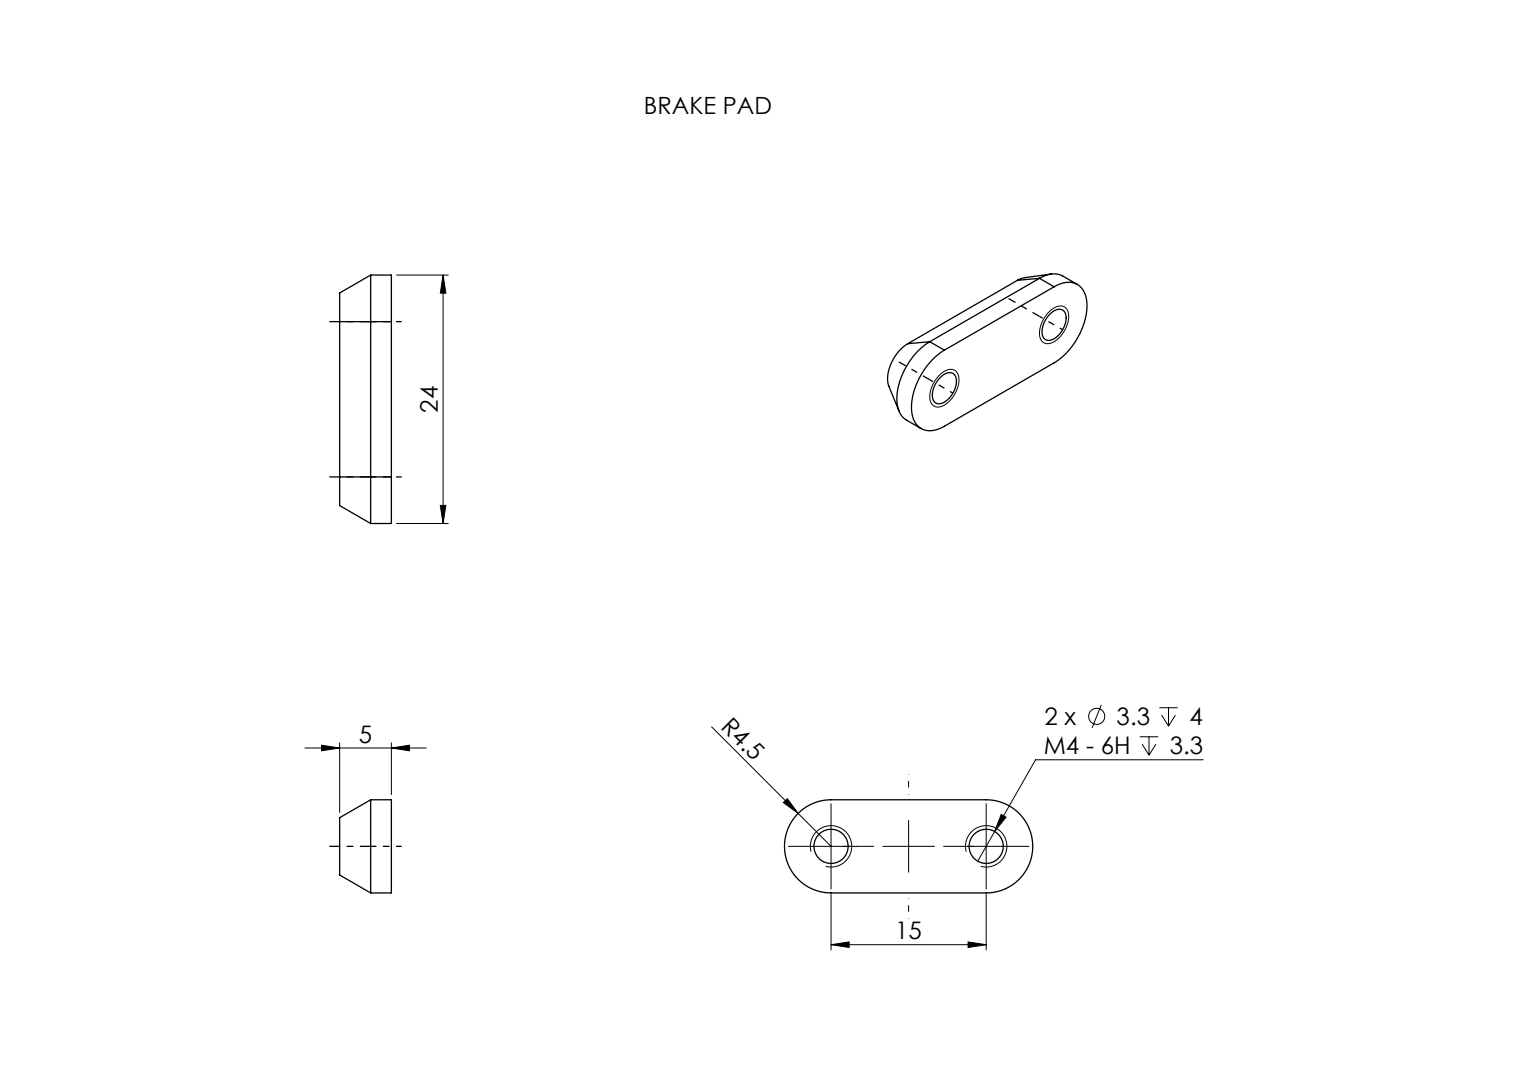
ISO-10303-21;
HEADER;
FILE_DESCRIPTION (('STEP AP214'),
    '1' );
FILE_NAME ('brake pad.step',
    '2026-10-08T05:45:04',
    ( '' ),
    ( '' ),
    'SwSTEP 2.0',
    'SolidWorks 2026',
    '' );
FILE_SCHEMA (( 'AUTOMOTIVE_DESIGN' ));
ENDSEC;

DATA;
#2=( LENGTH_UNIT ( ) NAMED_UNIT ( * ) SI_UNIT ( .MILLI., .METRE. ) );
#24=LINE ( 'NONE', #3426, #7602 ) ;
#25=FACE_OUTER_BOUND ( 'NONE', #10724, .T. ) ;
#72=( GEOMETRIC_REPRESENTATION_CONTEXT ( 3 ) GLOBAL_UNCERTAINTY_ASSIGNED_CONTEXT ( ( #3080 ) ) GLOBAL_UNIT_ASSIGNED_CONTEXT ( ( #8638, #7131, #1020 ) ) REPRESENTATION_CONTEXT ( 'NONE', 'WORKASPACE' ) );
#75=SHAPE_REPRESENTATION ( 'brake pad', ( #308 ), #6353 ) ;
#80=CARTESIAN_POINT ( 'NONE',  ( 24.49999999999999289, -3.999999999999986233, -4.999999999999992006 ) ) ;
#87=ADVANCED_FACE ( 'NONE', ( #5248 ), #2694, .F. ) ;
#161=ORIENTED_EDGE ( 'NONE', *, *, #5009, .F. ) ;
#193=ORIENTED_EDGE ( 'NONE', *, *, #720, .T. ) ;
#218=PRODUCT ( 'brake pad', 'brake pad', '', ( #1890 ) ) ;
#221=CIRCLE ( 'NONE', #5903, 1.649999999999998579 ) ;
#252=CONICAL_SURFACE ( 'NONE', #4877, 2.767949192431121919, 0.5235987755982963732 ) ;
#259=AXIS2_PLACEMENT_3D ( 'NONE', #6737, #6069, #4302 ) ;
#274=VECTOR ( 'NONE', #6744, 1000.000000000000000 ) ;
#281=VERTEX_POINT ( 'NONE', #1064 ) ;
#301=CARTESIAN_POINT ( 'NONE',  ( 24.49999999999999289, -3.999999999999986233, -9.499999999999991118 ) ) ;
#303=ORIENTED_EDGE ( 'NONE', *, *, #5009, .T. ) ;
#308=AXIS2_PLACEMENT_3D ( 'NONE', #6956, #4296, #9565 ) ;
#314=CARTESIAN_POINT ( 'NONE',  ( 27.50000000000001066, 0.5000000000000162093, 10.00000000000000888 ) ) ;
#336=FILL_AREA_STYLE ('',( #9671 ) ) ;
#356=FACE_OUTER_BOUND ( 'NONE', #2898, .T. ) ;
#358=EDGE_CURVE ( 'NONE', #6966, #10495, #2017, .T. ) ;
#363=DIRECTION ( 'NONE',  ( 0.000000000000000000, 0.000000000000000000, -1.000000000000000000 ) ) ;
#366=ORIENTED_EDGE ( 'NONE', *, *, #5633, .F. ) ;
#372=EDGE_CURVE ( 'NONE', #1417, #4847, #7538, .T. ) ;
#414=FACE_OUTER_BOUND ( 'NONE', #5327, .T. ) ;
#418=EDGE_CURVE ( 'NONE', #6185, #829, #4717, .T. ) ;
#431=ORIENTED_EDGE ( 'NONE', *, *, #9265, .T. ) ;
#465=CARTESIAN_POINT ( 'NONE',  ( 27.50000000000001066, -8.499999999999985789, -4.999999999999992006 ) ) ;
#486=EDGE_LOOP ( 'NONE', ( #10969, #5668, #5395 ) ) ;
#531=EDGE_LOOP ( 'NONE', ( #5767, #5211, #193 ) ) ;
#594=EDGE_LOOP ( 'NONE', ( #6389, #7026, #1992, #1296 ) ) ;
#605=CIRCLE ( 'NONE', #5598, 4.499999999999999112 ) ;
#653=DIRECTION ( 'NONE',  ( 1.000000000000000000, -0.000000000000000000, 1.156482317317871478E-16 ) ) ;
#675=CARTESIAN_POINT ( 'NONE',  ( 25.49999999999999645, -3.999999999999986233, -6.649999999999990585 ) ) ;
#686=LINE ( 'NONE', #7469, #1983 ) ;
#707=CARTESIAN_POINT ( 'NONE',  ( 27.50000000000001066, -3.999999999999986233, -4.999999999999992006 ) ) ;
#720=EDGE_CURVE ( 'NONE', #2294, #2160, #221, .T. ) ;
#723=DIRECTION ( 'NONE',  ( 1.000000000000000000, 0.000000000000000000, 0.000000000000000000 ) ) ;
#740=EDGE_CURVE ( 'NONE', #7218, #1417, #8677, .T. ) ;
#774=CIRCLE ( 'NONE', #5758, 4.499999999999999112 ) ;
#829=VERTEX_POINT ( 'NONE', #10864 ) ;
#848=CARTESIAN_POINT ( 'NONE',  ( 25.49999999999999645, -3.999999999999986233, -3.349999999999993427 ) ) ;
#860=DIRECTION ( 'NONE',  ( -1.156482317317871478E-16, 1.807003620809174139E-16, 1.000000000000000000 ) ) ;
#884=CARTESIAN_POINT ( 'NONE',  ( 25.49999999999999645, -3.999999999999983569, 10.00000000000000888 ) ) ;
#931=SHAPE_DEFINITION_REPRESENTATION ( #7149, #75 ) ;
#938=ADVANCED_FACE ( 'NONE', ( #10453 ), #10282, .T. ) ;
#967=AXIS2_PLACEMENT_3D ( 'NONE', #10328, #5168, #10996 ) ;
#969=DIRECTION ( 'NONE',  ( -1.156482317317871478E-16, 0.000000000000000000, 1.000000000000000000 ) ) ;
#993=CARTESIAN_POINT ( 'NONE',  ( 24.49999999999999289, -3.999999999999986233, -7.767949192431114369 ) ) ;
#997=DIRECTION ( 'NONE',  ( 0.000000000000000000, 0.000000000000000000, -1.000000000000000000 ) ) ;
#1020=( NAMED_UNIT ( * ) SI_UNIT ( $, .STERADIAN. ) SOLID_ANGLE_UNIT ( ) );
#1029=COLOUR_RGB ( '', 0.66274510, 0.83137255, 0.94901961) ;
#1036=AXIS2_PLACEMENT_3D ( 'NONE', #884, #10173, #2562 ) ;
#1038=DIRECTION ( 'NONE',  ( 0.5150380749100551547, 0.000000000000000000, -0.8571673007021116675 ) ) ;
#1064=CARTESIAN_POINT ( 'NONE',  ( 29.49999999999999645, -3.999999999999986233, -6.649999999999981704 ) ) ;
#1081=CIRCLE ( 'NONE', #4649, 2.767949192431121919 ) ;
#1153=ORIENTED_EDGE ( 'NONE', *, *, #10578, .F. ) ;
#1196=VECTOR ( 'NONE', #9291, 1000.000000000000000 ) ;
#1217=VECTOR ( 'NONE', #7964, 1000.000000000000114 ) ;
#1232=ADVANCED_BREP_SHAPE_REPRESENTATION ( '', ( #8973, #308 ), #6353 ) ;
#1245=DIRECTION ( 'NONE',  ( 0.000000000000000000, 0.000000000000000000, -1.000000000000000000 ) ) ;
#1275=DIRECTION ( 'NONE',  ( 1.000000000000000000, 6.098637220230963674E-17, 1.156482317317871478E-16 ) ) ;
#1288=VECTOR ( 'NONE', #2104, 1000.000000000000000 ) ;
#1289=EDGE_CURVE ( 'NONE', #829, #1417, #3766, .T. ) ;
#1296=ORIENTED_EDGE ( 'NONE', *, *, #9131, .F. ) ;
#1301=CARTESIAN_POINT ( 'NONE',  ( 29.49999999999999645, 0.5000000000000135447, -4.999999999999991118 ) ) ;
#1321=ADVANCED_FACE ( 'NONE', ( #414 ), #7150, .F. ) ;
#1334=VERTEX_POINT ( 'NONE', #314 ) ;
#1395=DIRECTION ( 'NONE',  ( 0.000000000000000000, 0.000000000000000000, 1.000000000000000000 ) ) ;
#1417=VERTEX_POINT ( 'NONE', #5545 ) ;
#1485=ORIENTED_EDGE ( 'NONE', *, *, #1289, .F. ) ;
#1496=VECTOR ( 'NONE', #2306, 1000.000000000000000 ) ;
#1541=VECTOR ( 'NONE', #2747, 1000.000000000000000 ) ;
#1555=CARTESIAN_POINT ( 'NONE',  ( 29.49999999999999645, -3.999999999999986233, -3.350000000000001421 ) ) ;
#1655=ORIENTED_EDGE ( 'NONE', *, *, #4757, .T. ) ;
#1686=CARTESIAN_POINT ( 'NONE',  ( 29.49999999999999645, -3.999999999999983569, 8.350000000000013856 ) ) ;
#1692=FACE_OUTER_BOUND ( 'NONE', #531, .T. ) ;
#1695=CONICAL_SURFACE ( 'NONE', #2228, 1.649999999999998579, 1.029744258676653423 ) ;
#1708=CARTESIAN_POINT ( 'NONE',  ( 29.49999999999999645, -3.999999999999983569, 11.64999999999999858 ) ) ;
#1725=ADVANCED_FACE ( 'NONE', ( #10146 ), #1763, .T. ) ;
#1727=FACE_OUTER_BOUND ( 'NONE', #10304, .T. ) ;
#1743=( GEOMETRIC_REPRESENTATION_CONTEXT ( 3 ) GLOBAL_UNCERTAINTY_ASSIGNED_CONTEXT ( ( #9535 ) ) GLOBAL_UNIT_ASSIGNED_CONTEXT ( ( #5567, #3731, #4682 ) ) REPRESENTATION_CONTEXT ( 'NONE', 'WORKASPACE' ) );
#1745=DIRECTION ( 'NONE',  ( 0.000000000000000000, 0.000000000000000000, -1.000000000000000000 ) ) ;
#1763=PLANE ( 'NONE',  #7963 ) ;
#1764=DIRECTION ( 'NONE',  ( 0.000000000000000000, 2.312964634635742464E-16, 1.000000000000000000 ) ) ;
#1769=EDGE_CURVE ( 'NONE', #4847, #3729, #24, .T. ) ;
#1854=ORIENTED_EDGE ( 'NONE', *, *, #4757, .F. ) ;
#1890=PRODUCT_CONTEXT ( 'NONE', #3230, 'mechanical' ) ;
#1901=DIRECTION ( 'NONE',  ( -0.8660254037844401509, 0.4999999999999974465, 0.000000000000000000 ) ) ;
#1911=DIRECTION ( 'NONE',  ( 0.000000000000000000, 0.000000000000000000, -1.000000000000000000 ) ) ;
#1914=DIRECTION ( 'NONE',  ( 0.000000000000000000, 0.000000000000000000, 1.000000000000000000 ) ) ;
#1915=CARTESIAN_POINT ( 'NONE',  ( 24.49999999999999289, -8.499999999999985789, -4.999999999999992006 ) ) ;
#1929=DIRECTION ( 'NONE',  ( -1.000000000000000000, -6.098637220230963674E-17, -1.156482317317871478E-16 ) ) ;
#1972=EDGE_CURVE ( 'NONE', #2160, #2294, #6718, .T. ) ;
#1983=VECTOR ( 'NONE', #10089, 1000.000000000000000 ) ;
#1992=ORIENTED_EDGE ( 'NONE', *, *, #4028, .T. ) ;
#1994=CARTESIAN_POINT ( 'NONE',  ( 27.50000000000001066, -8.499999999999984013, 10.00000000000001243 ) ) ;
#2015=ADVANCED_FACE ( 'NONE', ( #1727 ), #3351, .F. ) ;
#2017=LINE ( 'NONE', #1915, #5074 ) ;
#2062=LINE ( 'NONE', #7164, #5810 ) ;
#2072=AXIS2_PLACEMENT_3D ( 'NONE', #9436, #3758, #4652 ) ;
#2085=LINE ( 'NONE', #1301, #5488 ) ;
#2089=EDGE_CURVE ( 'NONE', #2779, #3903, #2085, .T. ) ;
#2104=DIRECTION ( 'NONE',  ( -1.156482317317871725E-16, 2.312964634635742464E-16, 1.000000000000000000 ) ) ;
#2133=ORIENTED_EDGE ( 'NONE', *, *, #2996, .T. ) ;
#2136=CARTESIAN_POINT ( 'NONE',  ( 27.50000000000000711, 0.5000000000000162093, 10.00000000000000888 ) ) ;
#2140=DIRECTION ( 'NONE',  ( 0.000000000000000000, 0.000000000000000000, -1.000000000000000000 ) ) ;
#2141=DIRECTION ( 'NONE',  ( 1.000000000000000000, -0.000000000000000000, 1.156482317317871478E-16 ) ) ;
#2160=VERTEX_POINT ( 'NONE', #3746 ) ;
#2184=DIRECTION ( 'NONE',  ( -1.000000000000000000, -6.098637220230963674E-17, -1.156482317317871478E-16 ) ) ;
#2228=AXIS2_PLACEMENT_3D ( 'NONE', #7641, #3363, #9240 ) ;
#2231=CARTESIAN_POINT ( 'NONE',  ( 24.49999999999999289, -3.999999999999986233, -4.999999999999992006 ) ) ;
#2242=DIRECTION ( 'NONE',  ( 0.000000000000000000, 0.000000000000000000, 1.000000000000000000 ) ) ;
#2251=AXIS2_PLACEMENT_3D ( 'NONE', #10250, #4308, #6026 ) ;
#2268=EDGE_CURVE ( 'NONE', #3729, #6185, #1081, .T. ) ;
#2294=VERTEX_POINT ( 'NONE', #675 ) ;
#2297=CARTESIAN_POINT ( 'NONE',  ( 24.49999999999999289, -8.499999999999985789, -4.999999999999992006 ) ) ;
#2306=DIRECTION ( 'NONE',  ( 1.000000000000000000, 6.098637220230963674E-17, 1.156482317317871478E-16 ) ) ;
#2331=ADVANCED_FACE ( 'NONE', ( #10074 ), #6055, .T. ) ;
#2360=ADVANCED_FACE ( 'NONE', ( #4245 ), #3127, .F. ) ;
#2376=ORIENTED_EDGE ( 'NONE', *, *, #4928, .T. ) ;
#2377=LINE ( 'NONE', #7492, #3098 ) ;
#2403=DIRECTION ( 'NONE',  ( -1.000000000000000000, -6.098637220230963674E-17, -1.156482317317871478E-16 ) ) ;
#2414=DIRECTION ( 'NONE',  ( 1.000000000000000000, -0.000000000000000000, 1.156482317317871478E-16 ) ) ;
#2461=ORIENTED_EDGE ( 'NONE', *, *, #2089, .F. ) ;
#2526=AXIS2_PLACEMENT_3D ( 'NONE', #10493, #8926, #363 ) ;
#2532=DIRECTION ( 'NONE',  ( -0.4999999999999978906, 0.8660254037844399289, -2.143152199010143228E-16 ) ) ;
#2538=CARTESIAN_POINT ( 'NONE',  ( 29.49999999999999645, -3.999999999999986233, -9.499999999999991118 ) ) ;
#2539=EDGE_CURVE ( 'NONE', #9740, #10159, #686, .T. ) ;
#2562=DIRECTION ( 'NONE',  ( 0.000000000000000000, 0.000000000000000000, -1.000000000000000000 ) ) ;
#2565=ORIENTED_EDGE ( 'NONE', *, *, #3436, .T. ) ;
#2567=ORIENTED_EDGE ( 'NONE', *, *, #418, .T. ) ;
#2601=CARTESIAN_POINT ( 'NONE',  ( 24.50857997860451931, -3.999999999999987121, -4.999999999999992006 ) ) ;
#2623=EDGE_CURVE ( 'NONE', #9740, #5796, #6861, .T. ) ;
#2668=EDGE_LOOP ( 'NONE', ( #5565, #9709, #10121, #7284 ) ) ;
#2678=DIRECTION ( 'NONE',  ( 0.000000000000000000, 0.000000000000000000, -1.000000000000000000 ) ) ;
#2688=ADVANCED_FACE ( 'NONE', ( #9748 ), #6356, .F. ) ;
#2694=CYLINDRICAL_SURFACE ( 'NONE', #259, 1.649999999999995248 ) ;
#2706=ADVANCED_FACE ( 'NONE', ( #8866 ), #5178, .T. ) ;
#2747=DIRECTION ( 'NONE',  ( 0.5150380749100549327, 1.049727191138617956E-16, 0.8571673007021118895 ) ) ;
#2754=CARTESIAN_POINT ( 'NONE',  ( 29.49999999999999645, -3.999999999999986233, -4.999999999999991118 ) ) ;
#2779=VERTEX_POINT ( 'NONE', #3908 ) ;
#2780=ORIENTED_EDGE ( 'NONE', *, *, #8807, .T. ) ;
#2814=PRESENTATION_STYLE_ASSIGNMENT (( #4529 ) ) ;
#2816=CARTESIAN_POINT ( 'NONE',  ( 27.50000000000001066, -3.999999999999986233, -9.499999999999991118 ) ) ;
#2822=CARTESIAN_POINT ( 'NONE',  ( 29.49999999999999645, -3.999999999999983569, 10.00000000000000888 ) ) ;
#2886=ORIENTED_EDGE ( 'NONE', *, *, #10498, .T. ) ;
#2898=EDGE_LOOP ( 'NONE', ( #4680, #4279, #4909, #1485 ) ) ;
#2943=EDGE_CURVE ( 'NONE', #9728, #2779, #4480, .T. ) ;
#2986=ORIENTED_EDGE ( 'NONE', *, *, #1972, .F. ) ;
#2996=EDGE_CURVE ( 'NONE', #5796, #10159, #3585, .T. ) ;
#3080=UNCERTAINTY_MEASURE_WITH_UNIT (LENGTH_MEASURE( 1.000000000000000082E-05 ), #8638, 'distance_accuracy_value', 'NONE');
#3089=EDGE_CURVE ( 'NONE', #7474, #2294, #5274, .T. ) ;
#3098=VECTOR ( 'NONE', #653, 1000.000000000000000 ) ;
#3108=ORIENTED_EDGE ( 'NONE', *, *, #720, .F. ) ;
#3110=ORIENTED_EDGE ( 'NONE', *, *, #2623, .F. ) ;
#3127=PLANE ( 'NONE',  #8017 ) ;
#3162=CARTESIAN_POINT ( 'NONE',  ( 24.49999999999999289, -3.999999999999986233, -4.999999999999992006 ) ) ;
#3166=DIRECTION ( 'NONE',  ( 1.000000000000000000, 0.000000000000000000, 0.000000000000000000 ) ) ;
#3186=ORIENTED_EDGE ( 'NONE', *, *, #3436, .F. ) ;
#3188=LINE ( 'NONE', #465, #6642 ) ;
#3230=APPLICATION_CONTEXT ( 'automotive_design' ) ;
#3235=DIRECTION ( 'NONE',  ( -1.000000000000000000, -6.098637220230963674E-17, -1.156482317317871478E-16 ) ) ;
#3271=STYLED_ITEM ( 'NONE', ( #2814 ), #8973 ) ;
#3320=VECTOR ( 'NONE', #6303, 1000.000000000000114 ) ;
#3351=CONICAL_SURFACE ( 'NONE', #1036, 1.649999999999998579, 1.029744258676653423 ) ;
#3363=DIRECTION ( 'NONE',  ( 1.000000000000000000, -0.000000000000000000, 1.156482317317871478E-16 ) ) ;
#3412=CARTESIAN_POINT ( 'NONE',  ( 24.49999999999999289, 0.5000000000000132117, -4.999999999999992006 ) ) ;
#3426=CARTESIAN_POINT ( 'NONE',  ( 24.49999999999999289, -1.232050807568863426, -4.999999999999992006 ) ) ;
#3430=FACE_OUTER_BOUND ( 'NONE', #486, .T. ) ;
#3436=EDGE_CURVE ( 'NONE', #10149, #4955, #6033, .T. ) ;
#3479=CIRCLE ( 'NONE', #4369, 1.649999999999989919 ) ;
#3495=EDGE_CURVE ( 'NONE', #9475, #5073, #3479, .T. ) ;
#3528=PLANE ( 'NONE',  #10429 ) ;
#3585=CIRCLE ( 'NONE', #6947, 1.649999999999998579 ) ;
#3676=EDGE_LOOP ( 'NONE', ( #10863, #2565, #9321, #10103 ) ) ;
#3680=CARTESIAN_POINT ( 'NONE',  ( 29.49999999999999645, -8.499999999999985789, -4.999999999999991118 ) ) ;
#3729=VERTEX_POINT ( 'NONE', #3958 ) ;
#3731=( NAMED_UNIT ( * ) PLANE_ANGLE_UNIT ( ) SI_UNIT ( $, .RADIAN. ) );
#3746=CARTESIAN_POINT ( 'NONE',  ( 25.49999999999999645, -3.999999999999986233, -3.349999999999993427 ) ) ;
#3758=DIRECTION ( 'NONE',  ( -0.4999999999999978906, -0.8660254037844399289, 1.424844972990615018E-16 ) ) ;
#3766=LINE ( 'NONE', #4659, #1288 ) ;
#3777=AXIS2_PLACEMENT_3D ( 'NONE', #6165, #6218, #2678 ) ;
#3797=LINE ( 'NONE', #2136, #8992 ) ;
#3820=AXIS2_PLACEMENT_3D ( 'NONE', #8689, #8737, #4523 ) ;
#3845=AXIS2_PLACEMENT_3D ( 'NONE', #2754, #9521, #4481 ) ;
#3851=ORIENTED_EDGE ( 'NONE', *, *, #4672, .F. ) ;
#3857=DIRECTION ( 'NONE',  ( 1.000000000000000000, 0.000000000000000000, 0.000000000000000000 ) ) ;
#3866=AXIS2_PLACEMENT_3D ( 'NONE', #7073, #4574, #1911 ) ;
#3875=ORIENTED_EDGE ( 'NONE', *, *, #358, .T. ) ;
#3890=DIRECTION ( 'NONE',  ( 1.000000000000000000, 0.000000000000000000, 0.000000000000000000 ) ) ;
#3903=VERTEX_POINT ( 'NONE', #8231 ) ;
#3908=CARTESIAN_POINT ( 'NONE',  ( 29.49999999999999645, 0.5000000000000163203, 10.00000000000000888 ) ) ;
#3920=LINE ( 'NONE', #7147, #7041 ) ;
#3941=ORIENTED_EDGE ( 'NONE', *, *, #2539, .T. ) ;
#3952=EDGE_LOOP ( 'NONE', ( #4222, #3108, #8056, #303 ) ) ;
#3958=CARTESIAN_POINT ( 'NONE',  ( 24.49999999999999289, -1.232050807568863426, -4.999999999999992006 ) ) ;
#3966=DIRECTION ( 'NONE',  ( 0.000000000000000000, 0.000000000000000000, -1.000000000000000000 ) ) ;
#3975=COLOUR_RGB ( '', 0.66274510, 0.83137255, 0.94901961) ;
#4028=EDGE_CURVE ( 'NONE', #3729, #10824, #3920, .T. ) ;
#4033=AXIS2_PLACEMENT_3D ( 'NONE', #2231, #7227, #10624 ) ;
#4057=AXIS2_PLACEMENT_3D ( 'NONE', #7619, #2141, #6162 ) ;
#4072=CARTESIAN_POINT ( 'NONE',  ( 24.49999999999998934, -3.999999999999983569, 10.00000000000000888 ) ) ;
#4091=CARTESIAN_POINT ( 'NONE',  ( 25.49999999999999645, -3.999999999999986233, -4.999999999999992006 ) ) ;
#4109=CARTESIAN_POINT ( 'NONE',  ( 27.50000000000001066, -3.999999999999986233, -4.999999999999992006 ) ) ;
#4171=ORIENTED_EDGE ( 'NONE', *, *, #2268, .T. ) ;
#4197=LINE ( 'NONE', #10977, #274 ) ;
#4216=ORIENTED_EDGE ( 'NONE', *, *, #7569, .F. ) ;
#4222=ORIENTED_EDGE ( 'NONE', *, *, #9998, .F. ) ;
#4245=FACE_OUTER_BOUND ( 'NONE', #5088, .T. ) ;
#4246=DIRECTION ( 'NONE',  ( 1.000000000000000000, -0.000000000000000000, 1.156482317317871478E-16 ) ) ;
#4266=CARTESIAN_POINT ( 'NONE',  ( 29.49999999999999645, -3.999999999999986233, -4.999999999999991118 ) ) ;
#4279=ORIENTED_EDGE ( 'NONE', *, *, #4527, .F. ) ;
#4296=DIRECTION ( 'NONE',  ( 0.000000000000000000, 0.000000000000000000, 1.000000000000000000 ) ) ;
#4302=DIRECTION ( 'NONE',  ( 0.000000000000000000, 0.000000000000000000, -1.000000000000000000 ) ) ;
#4308=DIRECTION ( 'NONE',  ( 1.000000000000000000, -0.000000000000000000, 1.156482317317871478E-16 ) ) ;
#4367=CARTESIAN_POINT ( 'NONE',  ( 29.49999999999999645, -3.999999999999986233, -4.999999999999991118 ) ) ;
#4369=AXIS2_PLACEMENT_3D ( 'NONE', #2822, #9581, #6194 ) ;
#4408=ORIENTED_EDGE ( 'NONE', *, *, #7649, .T. ) ;
#4424=DIRECTION ( 'NONE',  ( 6.098637220230961209E-17, -1.000000000000000000, 1.807003620809174139E-16 ) ) ;
#4425=ORIENTED_EDGE ( 'NONE', *, *, #418, .F. ) ;
#4430=FACE_OUTER_BOUND ( 'NONE', #6613, .T. ) ;
#4460=ADVANCED_FACE ( 'NONE', ( #356 ), #9384, .T. ) ;
#4480=CIRCLE ( 'NONE', #9606, 4.499999999999999112 ) ;
#4481=DIRECTION ( 'NONE',  ( -1.156482317317871478E-16, 0.000000000000000000, 1.000000000000000000 ) ) ;
#4495=CARTESIAN_POINT ( 'NONE',  ( 24.50857997860451931, -3.999999999999984457, 10.00000000000000888 ) ) ;
#4522=CARTESIAN_POINT ( 'NONE',  ( 29.49999999999999645, -3.999999999999986233, -4.999999999999991118 ) ) ;
#4523=DIRECTION ( 'NONE',  ( 0.000000000000000000, 0.000000000000000000, 1.000000000000000000 ) ) ;
#4525=ORIENTED_EDGE ( 'NONE', *, *, #10248, .F. ) ;
#4527=EDGE_CURVE ( 'NONE', #7218, #6966, #3188, .T. ) ;
#4529=SURFACE_STYLE_USAGE ( .BOTH. , #7084 ) ;
#4549=CARTESIAN_POINT ( 'NONE',  ( 29.49999999999999645, -8.499999999999984013, 10.00000000000001243 ) ) ;
#4574=DIRECTION ( 'NONE',  ( 1.000000000000000000, -0.000000000000000000, 1.156482317317871478E-16 ) ) ;
#4627=ORIENTED_EDGE ( 'NONE', *, *, #5270, .F. ) ;
#4649=AXIS2_PLACEMENT_3D ( 'NONE', #10961, #3235, #6676 ) ;
#4652=DIRECTION ( 'NONE',  ( 1.156482317317871725E-16, -2.312964634635742464E-16, -1.000000000000000000 ) ) ;
#4659=CARTESIAN_POINT ( 'NONE',  ( 24.49999999999999289, -6.767949192431104599, 10.00000000000001243 ) ) ;
#4661=ORIENTED_EDGE ( 'NONE', *, *, #2943, .T. ) ;
#4672=EDGE_CURVE ( 'NONE', #5073, #9475, #8103, .T. ) ;
#4680=ORIENTED_EDGE ( 'NONE', *, *, #5270, .T. ) ;
#4682=( NAMED_UNIT ( * ) SI_UNIT ( $, .STERADIAN. ) SOLID_ANGLE_UNIT ( ) );
#4692=ADVANCED_FACE ( 'NONE', ( #1692 ), #1695, .F. ) ;
#4703=CARTESIAN_POINT ( 'NONE',  ( 27.50000000000000711, 0.5000000000000162093, 10.00000000000000888 ) ) ;
#4708=CLOSED_SHELL ( 'NONE', ( #7780, #2015, #1321, #7507, #7568, #10629, #938, #2360, #8977, #5899, #8024, #4887, #1725, #2706, #2331, #4460, #4692, #2688, #8845, #87 ) ) ;
#4717=CIRCLE ( 'NONE', #8963, 2.767949192431121919 ) ;
#4718=DIRECTION ( 'NONE',  ( 1.000000000000000000, -0.000000000000000000, 1.156482317317871478E-16 ) ) ;
#4740=SURFACE_SIDE_STYLE ('',( #6337 ) ) ;
#4757=EDGE_CURVE ( 'NONE', #9093, #281, #10387, .T. ) ;
#4782=EDGE_LOOP ( 'NONE', ( #3186, #7899, #8361, #5934 ) ) ;
#4805=DIRECTION ( 'NONE',  ( 0.000000000000000000, 0.000000000000000000, 1.000000000000000000 ) ) ;
#4832=ORIENTED_EDGE ( 'NONE', *, *, #372, .F. ) ;
#4847=VERTEX_POINT ( 'NONE', #5471 ) ;
#4864=DIRECTION ( 'NONE',  ( 1.000000000000000000, -0.000000000000000000, 1.156482317317871478E-16 ) ) ;
#4875=MECHANICAL_DESIGN_GEOMETRIC_PRESENTATION_REPRESENTATION('',(#3271),#72);
#4877=AXIS2_PLACEMENT_3D ( 'NONE', #3162, #9002, #10715 ) ;
#4887=ADVANCED_FACE ( 'NONE', ( #8637, #7030, #4430 ), #6969, .F. ) ;
#4888=ORIENTED_EDGE ( 'NONE', *, *, #372, .T. ) ;
#4909=ORIENTED_EDGE ( 'NONE', *, *, #740, .T. ) ;
#4928=EDGE_CURVE ( 'NONE', #10824, #1334, #3797, .T. ) ;
#4955=VERTEX_POINT ( 'NONE', #2538 ) ;
#5009=EDGE_CURVE ( 'NONE', #281, #9093, #6475, .T. ) ;
#5073=VERTEX_POINT ( 'NONE', #9423 ) ;
#5074=VECTOR ( 'NONE', #6183, 1000.000000000000000 ) ;
#5088=EDGE_LOOP ( 'NONE', ( #6408, #9938, #3875, #5466 ) ) ;
#5127=AXIS2_PLACEMENT_3D ( 'NONE', #4522, #5461, #1914 ) ;
#5144=DIRECTION ( 'NONE',  ( 0.000000000000000000, -1.807003620809174139E-16, -1.000000000000000000 ) ) ;
#5168=DIRECTION ( 'NONE',  ( 1.000000000000000000, -0.000000000000000000, 1.156482317317871478E-16 ) ) ;
#5178=CONICAL_SURFACE ( 'NONE', #7657, 2.767949192431121919, 0.5235987755982963732 ) ;
#5211=ORIENTED_EDGE ( 'NONE', *, *, #3089, .T. ) ;
#5248=FACE_OUTER_BOUND ( 'NONE', #2668, .T. ) ;
#5249=LINE ( 'NONE', #848, #1541 ) ;
#5270=EDGE_CURVE ( 'NONE', #829, #6966, #5406, .T. ) ;
#5274=LINE ( 'NONE', #8660, #7843 ) ;
#5304=LINE ( 'NONE', #1686, #1196 ) ;
#5327=EDGE_LOOP ( 'NONE', ( #2986, #5909, #1655, #1153 ) ) ;
#5330=EDGE_CURVE ( 'NONE', #4955, #10495, #7237, .T. ) ;
#5385=CARTESIAN_POINT ( 'NONE',  ( 24.49999999999999289, 0.5000000000000132117, -4.999999999999992006 ) ) ;
#5395=ORIENTED_EDGE ( 'NONE', *, *, #1972, .T. ) ;
#5399=PRESENTATION_STYLE_ASSIGNMENT (( #8058 ) ) ;
#5406=LINE ( 'NONE', #7124, #1217 ) ;
#5425=LINE ( 'NONE', #4703, #3320 ) ;
#5461=DIRECTION ( 'NONE',  ( -1.000000000000000000, -6.098637220230963674E-17, -1.156482317317871478E-16 ) ) ;
#5466=ORIENTED_EDGE ( 'NONE', *, *, #8112, .T. ) ;
#5471=CARTESIAN_POINT ( 'NONE',  ( 24.49999999999998934, -1.232050807568860762, 10.00000000000000888 ) ) ;
#5474=FILL_AREA_STYLE ('',( #10472 ) ) ;
#5478=CARTESIAN_POINT ( 'NONE',  ( 29.49999999999999645, -3.999999999999986233, -4.999999999999991118 ) ) ;
#5483=ORIENTED_EDGE ( 'NONE', *, *, #1769, .T. ) ;
#5488=VECTOR ( 'NONE', #9747, 1000.000000000000000 ) ;
#5515=APPLICATION_CONTEXT ( 'automotive_design' ) ;
#5545=CARTESIAN_POINT ( 'NONE',  ( 24.49999999999999289, -6.767949192431106376, 10.00000000000001243 ) ) ;
#5565=ORIENTED_EDGE ( 'NONE', *, *, #7649, .F. ) ;
#5567=( LENGTH_UNIT ( ) NAMED_UNIT ( * ) SI_UNIT ( .MILLI., .METRE. ) );
#5582=CARTESIAN_POINT ( 'NONE',  ( 24.49999999999999289, -3.999999999999986233, -4.999999999999992006 ) ) ;
#5598=AXIS2_PLACEMENT_3D ( 'NONE', #707, #3166, #10833 ) ;
#5618=FACE_OUTER_BOUND ( 'NONE', #8349, .T. ) ;
#5633=EDGE_CURVE ( 'NONE', #1334, #4847, #5425, .T. ) ;
#5668=ORIENTED_EDGE ( 'NONE', *, *, #6000, .T. ) ;
#5688=DIRECTION ( 'NONE',  ( -6.098637220230959976E-17, 1.000000000000000000, -2.312964634635742464E-16 ) ) ;
#5758=AXIS2_PLACEMENT_3D ( 'NONE', #6435, #3890, #1395 ) ;
#5767=ORIENTED_EDGE ( 'NONE', *, *, #6000, .F. ) ;
#5796=VERTEX_POINT ( 'NONE', #7516 ) ;
#5798=DIRECTION ( 'NONE',  ( 0.000000000000000000, 0.000000000000000000, -1.000000000000000000 ) ) ;
#5810=VECTOR ( 'NONE', #10560, 1000.000000000000000 ) ;
#5844=ORIENTED_EDGE ( 'NONE', *, *, #5933, .F. ) ;
#5875=ORIENTED_EDGE ( 'NONE', *, *, #4028, .F. ) ;
#5882=CYLINDRICAL_SURFACE ( 'NONE', #967, 1.649999999999995248 ) ;
#5899=ADVANCED_FACE ( 'NONE', ( #6964 ), #3528, .F. ) ;
#5903=AXIS2_PLACEMENT_3D ( 'NONE', #10393, #4718, #997 ) ;
#5909=ORIENTED_EDGE ( 'NONE', *, *, #9998, .T. ) ;
#5933=EDGE_CURVE ( 'NONE', #10159, #5073, #5304, .T. ) ;
#5934=ORIENTED_EDGE ( 'NONE', *, *, #10248, .T. ) ;
#6000=EDGE_CURVE ( 'NONE', #7474, #2160, #5249, .T. ) ;
#6026=DIRECTION ( 'NONE',  ( 0.000000000000000000, 0.000000000000000000, -1.000000000000000000 ) ) ;
#6033=LINE ( 'NONE', #301, #8624 ) ;
#6034=EDGE_LOOP ( 'NONE', ( #6904, #4408, #6262, #5844 ) ) ;
#6045=FACE_OUTER_BOUND ( 'NONE', #6034, .T. ) ;
#6050=LINE ( 'NONE', #993, #8961 ) ;
#6055=CONICAL_SURFACE ( 'NONE', #8180, 2.767949192431121919, 0.5235987755982959291 ) ;
#6069=DIRECTION ( 'NONE',  ( 1.000000000000000000, -0.000000000000000000, 1.156482317317871478E-16 ) ) ;
#6115=AXIS2_PLACEMENT_3D ( 'NONE', #4091, #7708, #6805 ) ;
#6127=ORIENTED_EDGE ( 'NONE', *, *, #4928, .F. ) ;
#6162=DIRECTION ( 'NONE',  ( 0.000000000000000000, 0.000000000000000000, -1.000000000000000000 ) ) ;
#6165=CARTESIAN_POINT ( 'NONE',  ( 24.49999999999999289, -3.999999999999986233, -4.999999999999992006 ) ) ;
#6183=DIRECTION ( 'NONE',  ( 1.000000000000000000, 6.098637220230963674E-17, 1.156482317317871478E-16 ) ) ;
#6185=VERTEX_POINT ( 'NONE', #9624 ) ;
#6194=DIRECTION ( 'NONE',  ( 0.000000000000000000, 0.000000000000000000, -1.000000000000000000 ) ) ;
#6218=DIRECTION ( 'NONE',  ( 1.000000000000000000, 6.098637220230963674E-17, 1.156482317317871478E-16 ) ) ;
#6238=FACE_OUTER_BOUND ( 'NONE', #7070, .T. ) ;
#6262=ORIENTED_EDGE ( 'NONE', *, *, #3495, .T. ) ;
#6303=DIRECTION ( 'NONE',  ( -0.8660254037844398178, -0.4999999999999978351, 0.000000000000000000 ) ) ;
#6337=SURFACE_STYLE_FILL_AREA ( #336 ) ;
#6353=( GEOMETRIC_REPRESENTATION_CONTEXT ( 3 ) GLOBAL_UNCERTAINTY_ASSIGNED_CONTEXT ( ( #9242 ) ) GLOBAL_UNIT_ASSIGNED_CONTEXT ( ( #2, #9731, #10462 ) ) REPRESENTATION_CONTEXT ( 'NONE', 'WORKASPACE' ) );
#6356=CYLINDRICAL_SURFACE ( 'NONE', #8718, 1.649999999999994360 ) ;
#6389=ORIENTED_EDGE ( 'NONE', *, *, #9265, .F. ) ;
#6408=ORIENTED_EDGE ( 'NONE', *, *, #8807, .F. ) ;
#6435=CARTESIAN_POINT ( 'NONE',  ( 27.50000000000001066, -3.999999999999983569, 10.00000000000000888 ) ) ;
#6454=CONICAL_SURFACE ( 'NONE', #6115, 1.649999999999998579, 1.029744258676653423 ) ;
#6475=CIRCLE ( 'NONE', #7913, 1.649999999999989919 ) ;
#6507=CARTESIAN_POINT ( 'NONE',  ( 29.49999999999999645, -3.999999999999983569, 10.00000000000000888 ) ) ;
#6570=FACE_OUTER_BOUND ( 'NONE', #7638, .T. ) ;
#6587=ORIENTED_EDGE ( 'NONE', *, *, #6615, .T. ) ;
#6613=EDGE_LOOP ( 'NONE', ( #4525, #2461, #8996, #10753, #9685 ) ) ;
#6615=EDGE_CURVE ( 'NONE', #1334, #2779, #2062, .T. ) ;
#6642=VECTOR ( 'NONE', #10648, 1000.000000000000000 ) ;
#6667=ORIENTED_EDGE ( 'NONE', *, *, #8499, .F. ) ;
#6676=DIRECTION ( 'NONE',  ( 0.000000000000000000, 0.000000000000000000, 1.000000000000000000 ) ) ;
#6718=CIRCLE ( 'NONE', #4057, 1.649999999999998579 ) ;
#6737=CARTESIAN_POINT ( 'NONE',  ( 29.49999999999999645, -3.999999999999983569, 10.00000000000000888 ) ) ;
#6744=DIRECTION ( 'NONE',  ( 1.000000000000000000, -0.000000000000000000, 1.156482317317871478E-16 ) ) ;
#6803=CARTESIAN_POINT ( 'NONE',  ( 29.49999999999999645, -8.499999999999985789, -4.999999999999991118 ) ) ;
#6805=DIRECTION ( 'NONE',  ( 0.000000000000000000, 0.000000000000000000, -1.000000000000000000 ) ) ;
#6826=AXIS2_PLACEMENT_3D ( 'NONE', #4109, #8908, #10882 ) ;
#6861=LINE ( 'NONE', #6973, #8352 ) ;
#6889=STYLED_ITEM ( 'NONE', ( #5399 ), #1232 ) ;
#6904=ORIENTED_EDGE ( 'NONE', *, *, #2996, .F. ) ;
#6935=ORIENTED_EDGE ( 'NONE', *, *, #740, .F. ) ;
#6947=AXIS2_PLACEMENT_3D ( 'NONE', #9456, #4246, #1745 ) ;
#6949=ORIENTED_EDGE ( 'NONE', *, *, #7569, .T. ) ;
#6956=CARTESIAN_POINT ( 'NONE',  ( 0.000000000000000000, 0.000000000000000000, 0.000000000000000000 ) ) ;
#6964=FACE_OUTER_BOUND ( 'NONE', #9608, .T. ) ;
#6966=VERTEX_POINT ( 'NONE', #8433 ) ;
#6969=PLANE ( 'NONE',  #3845 ) ;
#6973=CARTESIAN_POINT ( 'NONE',  ( 25.49999999999999645, -3.999999999999983569, 11.65000000000000746 ) ) ;
#7003=EDGE_LOOP ( 'NONE', ( #3851, #8606 ) ) ;
#7026=ORIENTED_EDGE ( 'NONE', *, *, #2268, .F. ) ;
#7030=FACE_BOUND ( 'NONE', #9503, .T. ) ;
#7041=VECTOR ( 'NONE', #7305, 1000.000000000000114 ) ;
#7070=EDGE_LOOP ( 'NONE', ( #9225, #6949, #2780, #4661 ) ) ;
#7073=CARTESIAN_POINT ( 'NONE',  ( 25.49999999999999645, -3.999999999999983569, 10.00000000000000888 ) ) ;
#7084=SURFACE_SIDE_STYLE ('',( #7922 ) ) ;
#7086=DIRECTION ( 'NONE',  ( 0.000000000000000000, 0.000000000000000000, -1.000000000000000000 ) ) ;
#7124=CARTESIAN_POINT ( 'NONE',  ( 24.49999999999999289, -6.767949192431108152, -4.999999999999992006 ) ) ;
#7131=( NAMED_UNIT ( * ) PLANE_ANGLE_UNIT ( ) SI_UNIT ( $, .RADIAN. ) );
#7147=CARTESIAN_POINT ( 'NONE',  ( 24.49999999999999289, -1.232050807568863426, -4.999999999999992006 ) ) ;
#7149=PRODUCT_DEFINITION_SHAPE ( 'NONE', 'NONE',  #7765 ) ;
#7150=CYLINDRICAL_SURFACE ( 'NONE', #2526, 1.649999999999994360 ) ;
#7164=CARTESIAN_POINT ( 'NONE',  ( 24.49999999999999289, 0.5000000000000159872, 10.00000000000000888 ) ) ;
#7182=DIRECTION ( 'NONE',  ( -1.156482317317871478E-16, 1.807003620809174139E-16, 1.000000000000000000 ) ) ;
#7218=VERTEX_POINT ( 'NONE', #1994 ) ;
#7222=ORIENTED_EDGE ( 'NONE', *, *, #9123, .F. ) ;
#7227=DIRECTION ( 'NONE',  ( 1.000000000000000000, 6.098637220230963674E-17, 1.156482317317871478E-16 ) ) ;
#7232=DIRECTION ( 'NONE',  ( -1.000000000000000000, -6.098637220230963674E-17, -1.156482317317871478E-16 ) ) ;
#7237=CIRCLE ( 'NONE', #5127, 4.499999999999999112 ) ;
#7284=ORIENTED_EDGE ( 'NONE', *, *, #4672, .T. ) ;
#7302=CARTESIAN_POINT ( 'NONE',  ( 24.49999999999999289, -8.499999999999984013, 10.00000000000001243 ) ) ;
#7305=DIRECTION ( 'NONE',  ( 0.8660254037844398178, 0.4999999999999978351, 0.000000000000000000 ) ) ;
#7469=CARTESIAN_POINT ( 'NONE',  ( 25.49999999999999645, -3.999999999999983569, 8.350000000000010303 ) ) ;
#7474=VERTEX_POINT ( 'NONE', #2601 ) ;
#7492=CARTESIAN_POINT ( 'NONE',  ( 29.49999999999999645, -3.999999999999983569, 11.65000000000000391 ) ) ;
#7507=ADVANCED_FACE ( 'NONE', ( #3430 ), #6454, .F. ) ;
#7511=DIRECTION ( 'NONE',  ( 0.000000000000000000, 0.000000000000000000, -1.000000000000000000 ) ) ;
#7516=CARTESIAN_POINT ( 'NONE',  ( 25.49999999999999645, -3.999999999999983569, 11.65000000000000746 ) ) ;
#7529=CARTESIAN_POINT ( 'NONE',  ( 24.49999999999999289, -1.232050807568863426, -4.999999999999992895 ) ) ;
#7535=VECTOR ( 'NONE', #1275, 1000.000000000000000 ) ;
#7538=CIRCLE ( 'NONE', #3820, 2.767949192431121919 ) ;
#7568=ADVANCED_FACE ( 'NONE', ( #5618 ), #252, .T. ) ;
#7569=EDGE_CURVE ( 'NONE', #1334, #7218, #774, .T. ) ;
#7602=VECTOR ( 'NONE', #10198, 1000.000000000000000 ) ;
#7619=CARTESIAN_POINT ( 'NONE',  ( 25.49999999999999645, -3.999999999999986233, -4.999999999999992006 ) ) ;
#7638=EDGE_LOOP ( 'NONE', ( #3110, #3941, #2886 ) ) ;
#7641=CARTESIAN_POINT ( 'NONE',  ( 25.49999999999999645, -3.999999999999986233, -4.999999999999992006 ) ) ;
#7649=EDGE_CURVE ( 'NONE', #5796, #9475, #2377, .T. ) ;
#7657=AXIS2_PLACEMENT_3D ( 'NONE', #5582, #3857, #2140 ) ;
#7705=LINE ( 'NONE', #6803, #10376 ) ;
#7708=DIRECTION ( 'NONE',  ( 1.000000000000000000, -0.000000000000000000, 1.156482317317871478E-16 ) ) ;
#7716=CONICAL_SURFACE ( 'NONE', #8229, 1.649999999999998579, 1.029744258676653423 ) ;
#7760=PLANE ( 'NONE',  #8245 ) ;
#7765=PRODUCT_DEFINITION ( 'UNKNOWN', '', #8117, #10003 ) ;
#7780=ADVANCED_FACE ( 'NONE', ( #6045 ), #5882, .F. ) ;
#7843=VECTOR ( 'NONE', #1038, 1000.000000000000000 ) ;
#7865=DIRECTION ( 'NONE',  ( 1.000000000000000000, 6.098637220230963674E-17, 1.156482317317871478E-16 ) ) ;
#7899=ORIENTED_EDGE ( 'NONE', *, *, #9131, .T. ) ;
#7913=AXIS2_PLACEMENT_3D ( 'NONE', #4266, #10098, #10039 ) ;
#7922=SURFACE_STYLE_FILL_AREA ( #5474 ) ;
#7963=AXIS2_PLACEMENT_3D ( 'NONE', #7529, #2532, #860 ) ;
#7964=DIRECTION ( 'NONE',  ( 0.8660254037844398178, -0.4999999999999978351, 0.000000000000000000 ) ) ;
#8017=AXIS2_PLACEMENT_3D ( 'NONE', #2297, #5688, #8227 ) ;
#8024=ADVANCED_FACE ( 'NONE', ( #25 ), #7760, .T. ) ;
#8056=ORIENTED_EDGE ( 'NONE', *, *, #10578, .T. ) ;
#8058=SURFACE_STYLE_USAGE ( .BOTH. , #4740 ) ;
#8060=FACE_OUTER_BOUND ( 'NONE', #3676, .T. ) ;
#8074=CARTESIAN_POINT ( 'NONE',  ( 25.49999999999999645, -3.999999999999983569, 8.350000000000010303 ) ) ;
#8077=AXIS2_PLACEMENT_3D ( 'NONE', #4367, #2414, #5798 ) ;
#8103=CIRCLE ( 'NONE', #2251, 1.649999999999989919 ) ;
#8112=EDGE_CURVE ( 'NONE', #10495, #9728, #7705, .T. ) ;
#8117=PRODUCT_DEFINITION_FORMATION_WITH_SPECIFIED_SOURCE ( 'ANY', '', #218, .NOT_KNOWN. ) ;
#8118=CYLINDRICAL_SURFACE ( 'NONE', #4033, 4.499999999999999112 ) ;
#8133=DIRECTION ( 'NONE',  ( 1.000000000000000000, -0.000000000000000000, 1.156482317317871478E-16 ) ) ;
#8164=ORIENTED_EDGE ( 'NONE', *, *, #2089, .T. ) ;
#8180=AXIS2_PLACEMENT_3D ( 'NONE', #4072, #723, #7511 ) ;
#8223=ORIENTED_EDGE ( 'NONE', *, *, #2539, .F. ) ;
#8227=DIRECTION ( 'NONE',  ( 0.000000000000000000, 2.312964634635742464E-16, 1.000000000000000000 ) ) ;
#8229=AXIS2_PLACEMENT_3D ( 'NONE', #10856, #4864, #3966 ) ;
#8231=CARTESIAN_POINT ( 'NONE',  ( 29.49999999999999645, 0.5000000000000135447, -4.999999999999991118 ) ) ;
#8245=AXIS2_PLACEMENT_3D ( 'NONE', #80, #1929, #969 ) ;
#8321=ORIENTED_EDGE ( 'NONE', *, *, #2623, .T. ) ;
#8349=EDGE_LOOP ( 'NONE', ( #4425, #431, #7222, #4627 ) ) ;
#8352=VECTOR ( 'NONE', #10361, 1000.000000000000000 ) ;
#8361=ORIENTED_EDGE ( 'NONE', *, *, #8499, .T. ) ;
#8433=CARTESIAN_POINT ( 'NONE',  ( 27.50000000000001066, -8.499999999999985789, -4.999999999999992006 ) ) ;
#8480=ORIENTED_EDGE ( 'NONE', *, *, #1769, .F. ) ;
#8499=EDGE_CURVE ( 'NONE', #10824, #3903, #10606, .T. ) ;
#8501=CARTESIAN_POINT ( 'NONE',  ( 27.50000000000001066, 0.5000000000000134337, -4.999999999999992006 ) ) ;
#8606=ORIENTED_EDGE ( 'NONE', *, *, #3495, .F. ) ;
#8618=CIRCLE ( 'NONE', #8798, 4.499999999999999112 ) ;
#8624=VECTOR ( 'NONE', #9418, 1000.000000000000000 ) ;
#8637=FACE_BOUND ( 'NONE', #7003, .T. ) ;
#8638=( LENGTH_UNIT ( ) NAMED_UNIT ( * ) SI_UNIT ( .MILLI., .METRE. ) );
#8660=CARTESIAN_POINT ( 'NONE',  ( 25.49999999999999645, -3.999999999999986233, -6.649999999999990585 ) ) ;
#8668=MECHANICAL_DESIGN_GEOMETRIC_PRESENTATION_REPRESENTATION('',(#6889),#1743);
#8677=LINE ( 'NONE', #10455, #10169 ) ;
#8689=CARTESIAN_POINT ( 'NONE',  ( 24.49999999999998934, -3.999999999999983569, 10.00000000000000888 ) ) ;
#8718=AXIS2_PLACEMENT_3D ( 'NONE', #5478, #8133, #7086 ) ;
#8737=DIRECTION ( 'NONE',  ( -1.000000000000000000, -6.098637220230963674E-17, -1.156482317317871478E-16 ) ) ;
#8798=AXIS2_PLACEMENT_3D ( 'NONE', #9795, #2184, #2242 ) ;
#8807=EDGE_CURVE ( 'NONE', #7218, #9728, #9031, .T. ) ;
#8845=ADVANCED_FACE ( 'NONE', ( #6570 ), #7716, .F. ) ;
#8849=LINE ( 'NONE', #9510, #10960 ) ;
#8866=FACE_OUTER_BOUND ( 'NONE', #594, .T. ) ;
#8908=DIRECTION ( 'NONE',  ( 1.000000000000000000, 0.000000000000000000, 0.000000000000000000 ) ) ;
#8926=DIRECTION ( 'NONE',  ( 1.000000000000000000, -0.000000000000000000, 1.156482317317871478E-16 ) ) ;
#8961=VECTOR ( 'NONE', #9438, 1000.000000000000114 ) ;
#8963=AXIS2_PLACEMENT_3D ( 'NONE', #9788, #7232, #9901 ) ;
#8973=MANIFOLD_SOLID_BREP ( 'M4 Tapped Hole2', #4708 ) ;
#8977=ADVANCED_FACE ( 'NONE', ( #6238 ), #10581, .T. ) ;
#8992=VECTOR ( 'NONE', #7182, 1000.000000000000000 ) ;
#8996=ORIENTED_EDGE ( 'NONE', *, *, #2943, .F. ) ;
#9002=DIRECTION ( 'NONE',  ( 1.000000000000000000, 0.000000000000000000, 0.000000000000000000 ) ) ;
#9031=LINE ( 'NONE', #7302, #1496 ) ;
#9093=VERTEX_POINT ( 'NONE', #1555 ) ;
#9123=EDGE_CURVE ( 'NONE', #6966, #10149, #605, .T. ) ;
#9131=EDGE_CURVE ( 'NONE', #10149, #10824, #10202, .T. ) ;
#9225=ORIENTED_EDGE ( 'NONE', *, *, #6615, .F. ) ;
#9240=DIRECTION ( 'NONE',  ( 0.000000000000000000, 0.000000000000000000, -1.000000000000000000 ) ) ;
#9242=UNCERTAINTY_MEASURE_WITH_UNIT (LENGTH_MEASURE( 1.000000000000000082E-05 ), #2, 'distance_accuracy_value', 'NONE');
#9265=EDGE_CURVE ( 'NONE', #6185, #10149, #6050, .T. ) ;
#9291=DIRECTION ( 'NONE',  ( 1.000000000000000000, -0.000000000000000000, 1.156482317317871478E-16 ) ) ;
#9321=ORIENTED_EDGE ( 'NONE', *, *, #5330, .T. ) ;
#9368=EDGE_LOOP ( 'NONE', ( #366, #6127, #5875, #8480 ) ) ;
#9384=PLANE ( 'NONE',  #2072 ) ;
#9418=DIRECTION ( 'NONE',  ( 1.000000000000000000, 6.098637220230963674E-17, 1.156482317317871478E-16 ) ) ;
#9423=CARTESIAN_POINT ( 'NONE',  ( 29.49999999999999645, -3.999999999999983569, 8.350000000000019185 ) ) ;
#9436=CARTESIAN_POINT ( 'NONE',  ( 24.49999999999999289, -6.767949192431108152, -4.999999999999991118 ) ) ;
#9438=DIRECTION ( 'NONE',  ( 0.8660254037844398178, 0.000000000000000000, -0.4999999999999978351 ) ) ;
#9456=CARTESIAN_POINT ( 'NONE',  ( 25.49999999999999645, -3.999999999999983569, 10.00000000000000888 ) ) ;
#9475=VERTEX_POINT ( 'NONE', #1708 ) ;
#9484=AXIS2_PLACEMENT_3D ( 'NONE', #10526, #7865, #1245 ) ;
#9503=EDGE_LOOP ( 'NONE', ( #161, #1854 ) ) ;
#9510=CARTESIAN_POINT ( 'NONE',  ( 29.49999999999999645, -3.999999999999986233, -6.649999999999986144 ) ) ;
#9521=DIRECTION ( 'NONE',  ( -1.000000000000000000, -6.098637220230963674E-17, -1.156482317317871478E-16 ) ) ;
#9535=UNCERTAINTY_MEASURE_WITH_UNIT (LENGTH_MEASURE( 1.000000000000000082E-05 ), #5567, 'distance_accuracy_value', 'NONE');
#9565=DIRECTION ( 'NONE',  ( 1.000000000000000000, 0.000000000000000000, 0.000000000000000000 ) ) ;
#9567=DIRECTION ( 'NONE',  ( 1.000000000000000000, -0.000000000000000000, 1.156482317317871478E-16 ) ) ;
#9581=DIRECTION ( 'NONE',  ( 1.000000000000000000, -0.000000000000000000, 1.156482317317871478E-16 ) ) ;
#9606=AXIS2_PLACEMENT_3D ( 'NONE', #6507, #2403, #4805 ) ;
#9608=EDGE_LOOP ( 'NONE', ( #6667, #2376, #6587, #8164 ) ) ;
#9615=SHAPE_REPRESENTATION_RELATIONSHIP ( 'NONE' , 'NONE' ,  #75, #1232 ) ;
#9624=CARTESIAN_POINT ( 'NONE',  ( 24.49999999999999289, -3.999999999999986233, -7.767949192431114369 ) ) ;
#9671=FILL_AREA_STYLE_COLOUR ( '', #1029 ) ;
#9685=ORIENTED_EDGE ( 'NONE', *, *, #5330, .F. ) ;
#9709=ORIENTED_EDGE ( 'NONE', *, *, #10498, .F. ) ;
#9728=VERTEX_POINT ( 'NONE', #4549 ) ;
#9731=( NAMED_UNIT ( * ) PLANE_ANGLE_UNIT ( ) SI_UNIT ( $, .RADIAN. ) );
#9740=VERTEX_POINT ( 'NONE', #4495 ) ;
#9747=DIRECTION ( 'NONE',  ( -0.000000000000000000, -1.807003620809174139E-16, -1.000000000000000000 ) ) ;
#9748=FACE_OUTER_BOUND ( 'NONE', #3952, .T. ) ;
#9788=CARTESIAN_POINT ( 'NONE',  ( 24.49999999999999289, -3.999999999999986233, -4.999999999999992006 ) ) ;
#9795=CARTESIAN_POINT ( 'NONE',  ( 29.49999999999999645, -3.999999999999986233, -4.999999999999991118 ) ) ;
#9901=DIRECTION ( 'NONE',  ( 0.000000000000000000, 0.000000000000000000, 1.000000000000000000 ) ) ;
#9935=ORIENTED_EDGE ( 'NONE', *, *, #1289, .T. ) ;
#9938=ORIENTED_EDGE ( 'NONE', *, *, #4527, .T. ) ;
#9998=EDGE_CURVE ( 'NONE', #2160, #9093, #4197, .T. ) ;
#10003=PRODUCT_DEFINITION_CONTEXT ( 'detailed design', #5515, 'design' ) ;
#10039=DIRECTION ( 'NONE',  ( 0.000000000000000000, 0.000000000000000000, -1.000000000000000000 ) ) ;
#10074=FACE_OUTER_BOUND ( 'NONE', #10737, .T. ) ;
#10089=DIRECTION ( 'NONE',  ( 0.5150380749100551547, 0.000000000000000000, -0.8571673007021116675 ) ) ;
#10098=DIRECTION ( 'NONE',  ( 1.000000000000000000, -0.000000000000000000, 1.156482317317871478E-16 ) ) ;
#10103=ORIENTED_EDGE ( 'NONE', *, *, #358, .F. ) ;
#10121=ORIENTED_EDGE ( 'NONE', *, *, #5933, .T. ) ;
#10146=FACE_OUTER_BOUND ( 'NONE', #9368, .T. ) ;
#10149=VERTEX_POINT ( 'NONE', #2816 ) ;
#10159=VERTEX_POINT ( 'NONE', #8074 ) ;
#10169=VECTOR ( 'NONE', #1901, 1000.000000000000227 ) ;
#10173=DIRECTION ( 'NONE',  ( 1.000000000000000000, -0.000000000000000000, 1.156482317317871478E-16 ) ) ;
#10198=DIRECTION ( 'NONE',  ( 1.156482317317871478E-16, -1.807003620809174139E-16, -1.000000000000000000 ) ) ;
#10202=CIRCLE ( 'NONE', #6826, 4.499999999999999112 ) ;
#10248=EDGE_CURVE ( 'NONE', #3903, #4955, #8618, .T. ) ;
#10250=CARTESIAN_POINT ( 'NONE',  ( 29.49999999999999645, -3.999999999999983569, 10.00000000000000888 ) ) ;
#10252=CIRCLE ( 'NONE', #3866, 1.649999999999998579 ) ;
#10282=CYLINDRICAL_SURFACE ( 'NONE', #3777, 4.499999999999999112 ) ;
#10304=EDGE_LOOP ( 'NONE', ( #8223, #8321, #2133 ) ) ;
#10328=CARTESIAN_POINT ( 'NONE',  ( 29.49999999999999645, -3.999999999999983569, 10.00000000000000888 ) ) ;
#10361=DIRECTION ( 'NONE',  ( 0.5150380749100549327, 1.049727191138617956E-16, 0.8571673007021118895 ) ) ;
#10376=VECTOR ( 'NONE', #1764, 1000.000000000000000 ) ;
#10387=CIRCLE ( 'NONE', #8077, 1.649999999999989919 ) ;
#10393=CARTESIAN_POINT ( 'NONE',  ( 25.49999999999999645, -3.999999999999986233, -4.999999999999992006 ) ) ;
#10429=AXIS2_PLACEMENT_3D ( 'NONE', #3412, #4424, #5144 ) ;
#10453=FACE_OUTER_BOUND ( 'NONE', #4782, .T. ) ;
#10455=CARTESIAN_POINT ( 'NONE',  ( 27.50000000000001066, -8.499999999999982236, 10.00000000000001243 ) ) ;
#10462=( NAMED_UNIT ( * ) SI_UNIT ( $, .STERADIAN. ) SOLID_ANGLE_UNIT ( ) );
#10472=FILL_AREA_STYLE_COLOUR ( '', #3975 ) ;
#10493=CARTESIAN_POINT ( 'NONE',  ( 29.49999999999999645, -3.999999999999986233, -4.999999999999991118 ) ) ;
#10495=VERTEX_POINT ( 'NONE', #3680 ) ;
#10498=EDGE_CURVE ( 'NONE', #10159, #5796, #10252, .T. ) ;
#10526=CARTESIAN_POINT ( 'NONE',  ( 24.49999999999999289, -3.999999999999983569, 10.00000000000000888 ) ) ;
#10560=DIRECTION ( 'NONE',  ( 1.000000000000000000, 6.098637220230963674E-17, 1.156482317317871478E-16 ) ) ;
#10578=EDGE_CURVE ( 'NONE', #2294, #281, #8849, .T. ) ;
#10581=CYLINDRICAL_SURFACE ( 'NONE', #9484, 4.499999999999999112 ) ;
#10606=LINE ( 'NONE', #5385, #7535 ) ;
#10624=DIRECTION ( 'NONE',  ( 0.000000000000000000, 0.000000000000000000, -1.000000000000000000 ) ) ;
#10629=ADVANCED_FACE ( 'NONE', ( #8060 ), #8118, .T. ) ;
#10648=DIRECTION ( 'NONE',  ( 1.156482317317871725E-16, -2.312964634635742464E-16, -1.000000000000000000 ) ) ;
#10691=ORIENTED_EDGE ( 'NONE', *, *, #5633, .T. ) ;
#10715=DIRECTION ( 'NONE',  ( 0.000000000000000000, 0.000000000000000000, -1.000000000000000000 ) ) ;
#10724=EDGE_LOOP ( 'NONE', ( #4171, #2567, #9935, #4888, #5483 ) ) ;
#10737=EDGE_LOOP ( 'NONE', ( #10691, #4832, #6935, #4216 ) ) ;
#10753=ORIENTED_EDGE ( 'NONE', *, *, #8112, .F. ) ;
#10824=VERTEX_POINT ( 'NONE', #8501 ) ;
#10833=DIRECTION ( 'NONE',  ( 0.000000000000000000, 0.000000000000000000, 1.000000000000000000 ) ) ;
#10856=CARTESIAN_POINT ( 'NONE',  ( 25.49999999999999645, -3.999999999999983569, 10.00000000000000888 ) ) ;
#10863=ORIENTED_EDGE ( 'NONE', *, *, #9123, .T. ) ;
#10864=CARTESIAN_POINT ( 'NONE',  ( 24.49999999999999289, -6.767949192431108152, -4.999999999999992006 ) ) ;
#10882=DIRECTION ( 'NONE',  ( 0.000000000000000000, 0.000000000000000000, 1.000000000000000000 ) ) ;
#10960=VECTOR ( 'NONE', #9567, 1000.000000000000000 ) ;
#10961=CARTESIAN_POINT ( 'NONE',  ( 24.49999999999999289, -3.999999999999986233, -4.999999999999992006 ) ) ;
#10969=ORIENTED_EDGE ( 'NONE', *, *, #3089, .F. ) ;
#10977=CARTESIAN_POINT ( 'NONE',  ( 29.49999999999999645, -3.999999999999986233, -3.349999999999996980 ) ) ;
#10996=DIRECTION ( 'NONE',  ( 0.000000000000000000, 0.000000000000000000, -1.000000000000000000 ) ) ;
ENDSEC;
END-ISO-10303-21;
